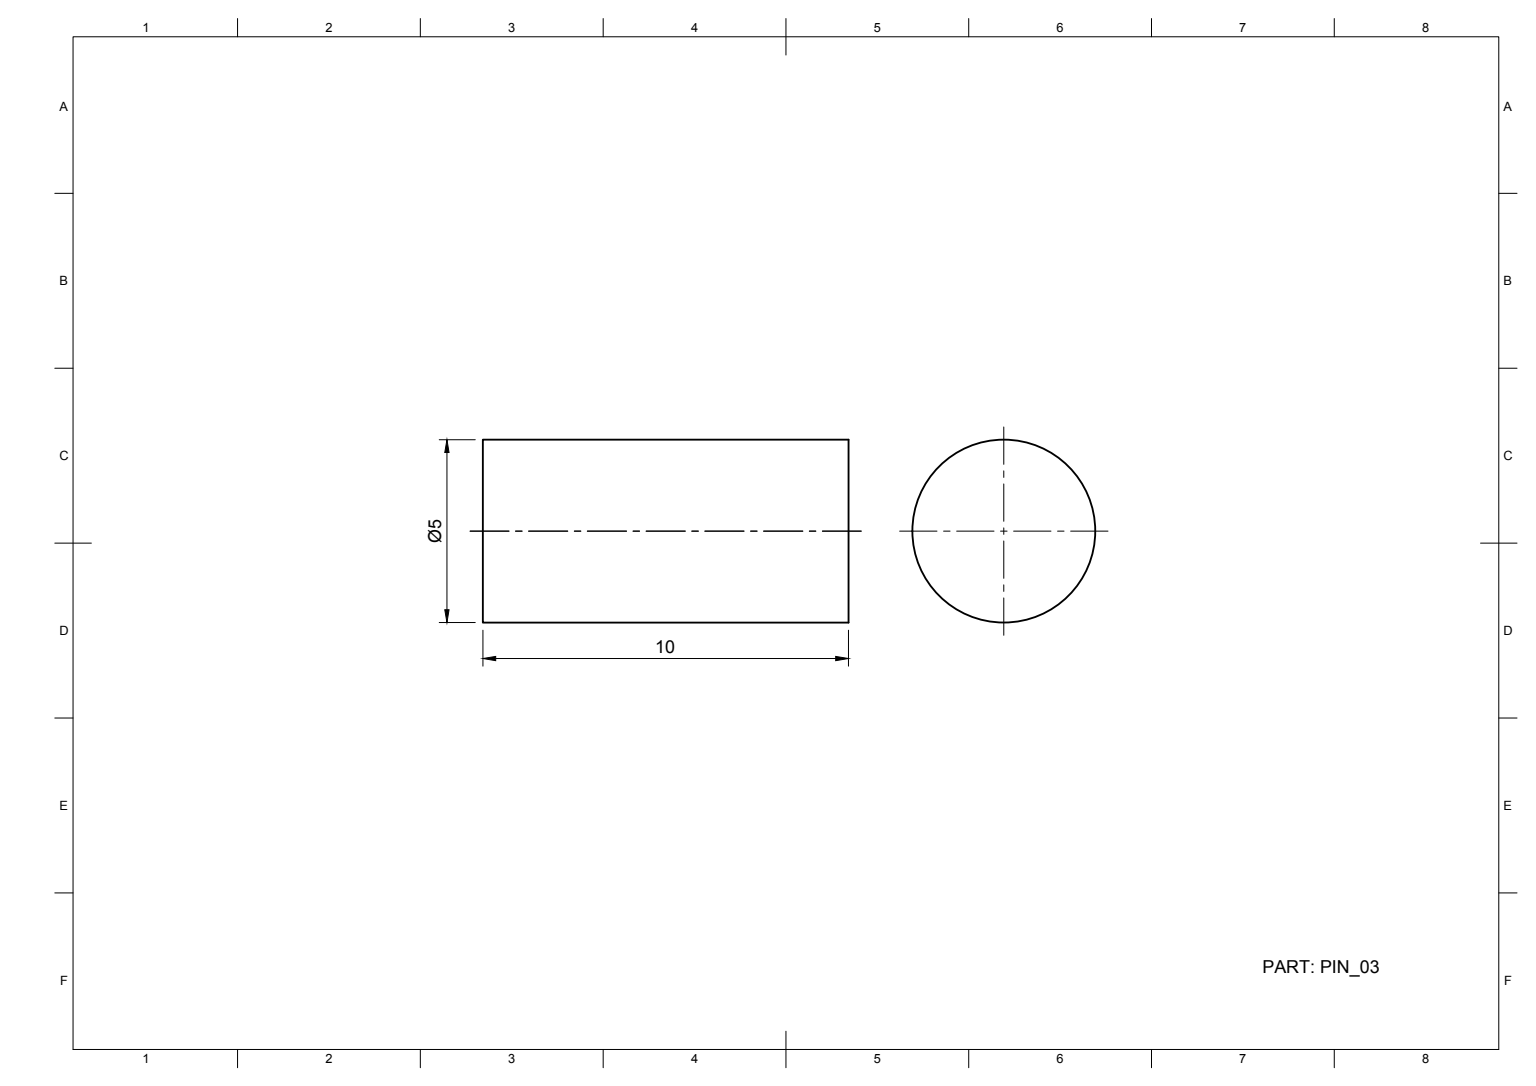
ISO-10303-21;
HEADER;
/* Generated by software containing ST-Developer
 * from STEP Tools, Inc. (www.steptools.com) 
 */

FILE_DESCRIPTION(
/* description */ (''),
/* implementation_level */ '2;1');

FILE_NAME(
/* name */ 'Pin_03.step',
/* time_stamp */ '2026-09-20T21:52:48+06:00',
/* author */ (''),
/* organization */ (''),
/* preprocessor_version */ 'ST-DEVELOPER v20.2',
/* originating_system */ 'Autodesk Translation Framework v15.15.0.0',
/* authorisation */ '');

FILE_SCHEMA (('AUTOMOTIVE_DESIGN { 1 0 10303 214 3 1 1 }'));
ENDSEC;

DATA;
#10=MECHANICAL_DESIGN_GEOMETRIC_PRESENTATION_REPRESENTATION('',(#65),#2203);
#49=SHAPE_REPRESENTATION_RELATIONSHIP('SRR','None',#2241,#57);
#57=ADVANCED_BREP_SHAPE_REPRESENTATION('',(#73),#2201);
#65=STYLED_ITEM('',(#2286),#73);
#73=MANIFOLD_SOLID_BREP('Pin_03',#1232);
#131=CIRCLE('',#1436,2.5);
#132=CIRCLE('',#1438,2.5);
#158=CYLINDRICAL_SURFACE('',#1437,2.5);
#223=FACE_OUTER_BOUND('',#304,.T.);
#224=FACE_OUTER_BOUND('',#305,.T.);
#225=FACE_OUTER_BOUND('',#306,.T.);
#304=EDGE_LOOP('',(#1094));
#305=EDGE_LOOP('',(#1095,#1096,#1097,#1098));
#306=EDGE_LOOP('',(#1099));
#420=LINE('',#2158,#530);
#530=VECTOR('',#1794,2.5);
#632=VERTEX_POINT('',#2154);
#633=VERTEX_POINT('',#2157);
#787=EDGE_CURVE('',#632,#632,#131,.T.);
#788=EDGE_CURVE('',#632,#633,#420,.T.);
#789=EDGE_CURVE('',#633,#633,#132,.T.);
#1094=ORIENTED_EDGE('',*,*,#787,.T.);
#1095=ORIENTED_EDGE('',*,*,#787,.F.);
#1096=ORIENTED_EDGE('',*,*,#788,.T.);
#1097=ORIENTED_EDGE('',*,*,#789,.T.);
#1098=ORIENTED_EDGE('',*,*,#788,.F.);
#1099=ORIENTED_EDGE('',*,*,#789,.F.);
#1153=PLANE('',#1435);
#1154=PLANE('',#1439);
#1219=ADVANCED_FACE('',(#223),#1153,.T.);
#1220=ADVANCED_FACE('',(#224),#158,.T.);
#1221=ADVANCED_FACE('',(#225),#1154,.T.);
#1232=CLOSED_SHELL('',(#1219,#1220,#1221));
#1434=AXIS2_PLACEMENT_3D('',#2152,#1786,#1787);
#1435=AXIS2_PLACEMENT_3D('',#2153,#1788,#1789);
#1436=AXIS2_PLACEMENT_3D('',#2155,#1790,#1791);
#1437=AXIS2_PLACEMENT_3D('',#2156,#1792,#1793);
#1438=AXIS2_PLACEMENT_3D('',#2159,#1795,#1796);
#1439=AXIS2_PLACEMENT_3D('',#2160,#1797,#1798);
#1786=DIRECTION('axis',(0.,0.,1.));
#1787=DIRECTION('refdir',(1.,0.,0.));
#1788=DIRECTION('center_axis',(0.,-1.,0.));
#1789=DIRECTION('ref_axis',(1.,0.,0.));
#1790=DIRECTION('center_axis',(0.,-1.,0.));
#1791=DIRECTION('ref_axis',(1.,0.,0.));
#1792=DIRECTION('center_axis',(0.,-1.,0.));
#1793=DIRECTION('ref_axis',(1.,0.,0.));
#1794=DIRECTION('',(0.,1.,0.));
#1795=DIRECTION('center_axis',(0.,-1.,0.));
#1796=DIRECTION('ref_axis',(1.,0.,0.));
#1797=DIRECTION('center_axis',(0.,1.,0.));
#1798=DIRECTION('ref_axis',(0.,0.,1.));
#2152=CARTESIAN_POINT('',(0.,0.,0.));
#2153=CARTESIAN_POINT('Origin',(0.,-5.,26.3));
#2154=CARTESIAN_POINT('',(-2.5,-5.,26.3));
#2155=CARTESIAN_POINT('Origin',(0.,-5.,26.3));
#2156=CARTESIAN_POINT('Origin',(0.,3.,26.3));
#2157=CARTESIAN_POINT('',(-2.5,5.,26.3));
#2158=CARTESIAN_POINT('',(-2.5,3.,26.3));
#2159=CARTESIAN_POINT('Origin',(0.,5.,26.3));
#2160=CARTESIAN_POINT('Origin',(0.,5.,50.));
#2191=UNCERTAINTY_MEASURE_WITH_UNIT(LENGTH_MEASURE(0.01),#2204,
'DISTANCE_ACCURACY_VALUE',
'Maximum model space distance between geometric entities at asserted c
onnectivities');
#2193=UNCERTAINTY_MEASURE_WITH_UNIT(LENGTH_MEASURE(0.01),#2204,
'DISTANCE_ACCURACY_VALUE',
'Maximum model space distance between geometric entities at asserted c
onnectivities');
#2201=(
GEOMETRIC_REPRESENTATION_CONTEXT(3)
GLOBAL_UNCERTAINTY_ASSIGNED_CONTEXT((#2191))
GLOBAL_UNIT_ASSIGNED_CONTEXT((#2204,#2206,#2207))
REPRESENTATION_CONTEXT('','3D')
);
#2203=(
GEOMETRIC_REPRESENTATION_CONTEXT(3)
GLOBAL_UNCERTAINTY_ASSIGNED_CONTEXT((#2193))
GLOBAL_UNIT_ASSIGNED_CONTEXT((#2204,#2206,#2207))
REPRESENTATION_CONTEXT('','3D')
);
#2204=(
LENGTH_UNIT()
NAMED_UNIT(*)
SI_UNIT(.MILLI.,.METRE.)
);
#2206=(
NAMED_UNIT(*)
PLANE_ANGLE_UNIT()
SI_UNIT($,.RADIAN.)
);
#2207=(
NAMED_UNIT(*)
SI_UNIT($,.STERADIAN.)
SOLID_ANGLE_UNIT()
);
#2215=SHAPE_DEFINITION_REPRESENTATION(#2224,#2241);
#2224=PRODUCT_DEFINITION_SHAPE('',$,#2251);
#2241=SHAPE_REPRESENTATION('',(#1434),#2201);
#2243=PRODUCT_DEFINITION_CONTEXT('part definition',#2272,'design');
#2251=PRODUCT_DEFINITION('Pin_03','Pin_03',#2260,#2243);
#2260=PRODUCT_DEFINITION_FORMATION('',$,#2281);
#2272=APPLICATION_CONTEXT(
'Core Data for Automotive Mechanical Design Process');
#2273=PRODUCT_CONTEXT('part definition',#2272,'mechanical');
#2281=PRODUCT('Pin_03','Pin_03',$,(#2273));
#2286=PRESENTATION_STYLE_ASSIGNMENT((#2290));
#2290=SURFACE_STYLE_USAGE(.BOTH.,#2294);
#2294=SURFACE_SIDE_STYLE('',(#2298));
#2298=SURFACE_STYLE_FILL_AREA(#2302);
#2302=FILL_AREA_STYLE('Surface - Matte',(#2306));
#2306=FILL_AREA_STYLE_COLOUR('Surface - Matte',#2310);
#2310=COLOUR_RGB('Surface - Matte', 0.31764706, 0.68627451, 0.89019608);
ENDSEC;
END-ISO-10303-21;
